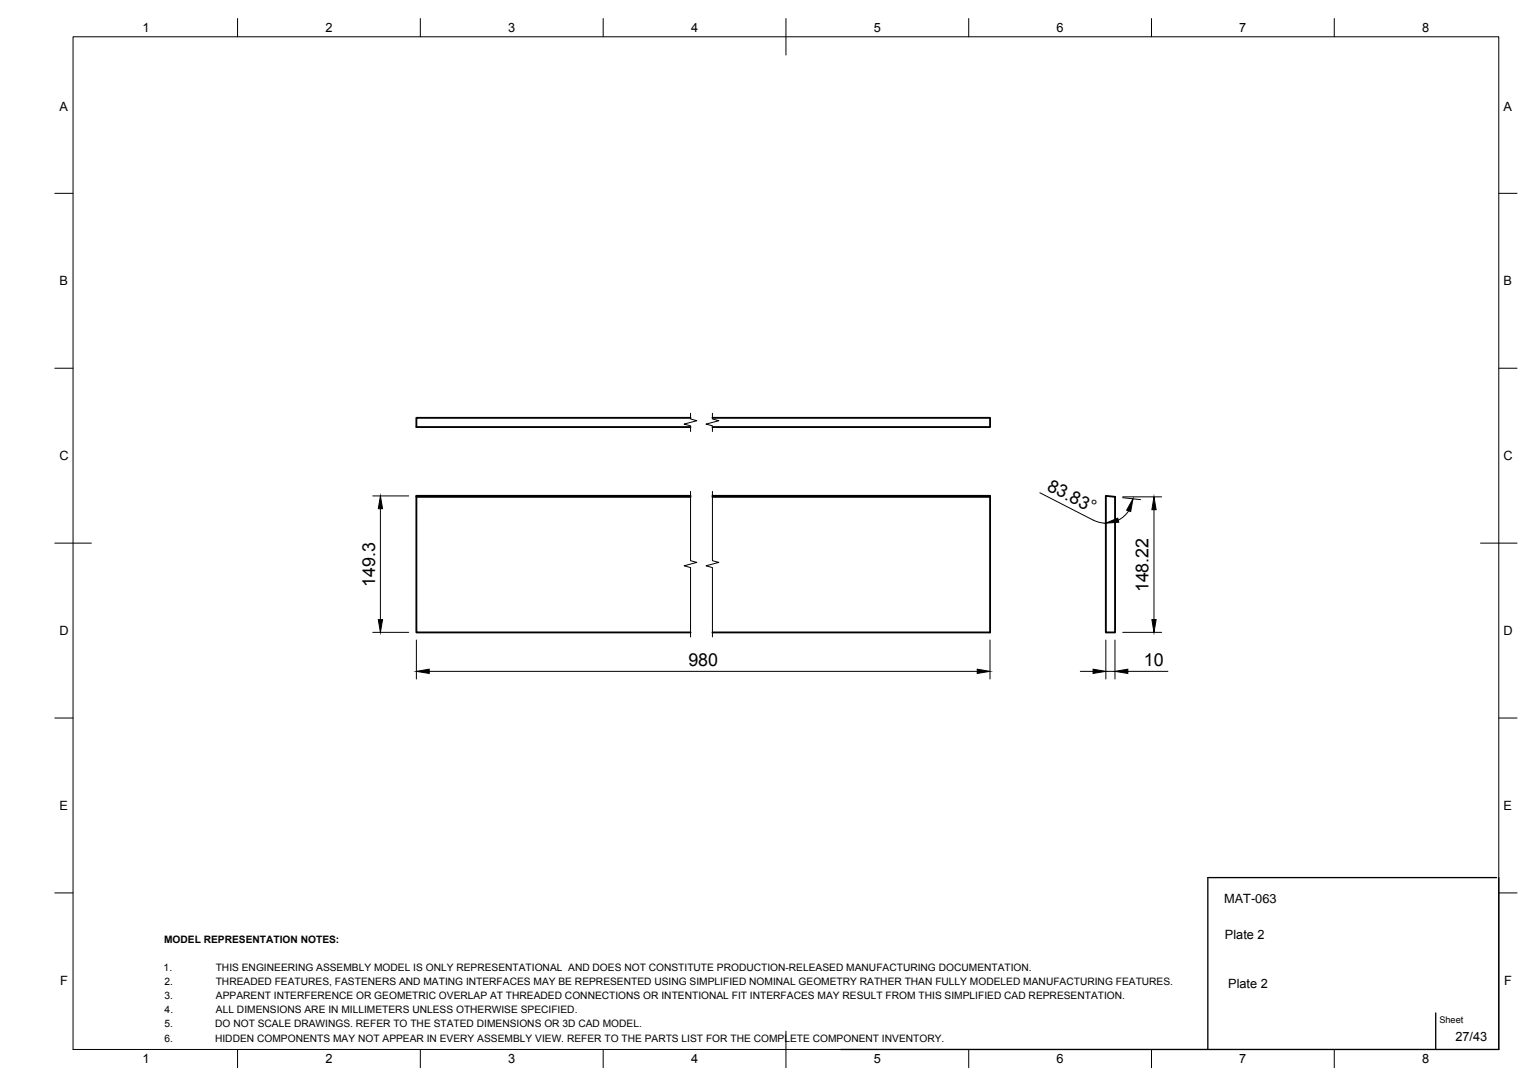
ISO-10303-21;
HEADER;
/* Generated by software containing ST-Developer
 * from STEP Tools, Inc. (www.steptools.com) 
 */

FILE_DESCRIPTION(
/* description */ (''),
/* implementation_level */ '2;1');

FILE_NAME(
/* name */ 'Plate 2.step',
/* time_stamp */ '2026-10-24T09:43:01-07:00',
/* author */ (''),
/* organization */ (''),
/* preprocessor_version */ 'ST-DEVELOPER v20.2',
/* originating_system */ 'Autodesk Translation Framework v15.15.0.0',
/* authorisation */ '');

FILE_SCHEMA (('AUTOMOTIVE_DESIGN { 1 0 10303 214 3 1 1 }'));
ENDSEC;

DATA;
#10=MECHANICAL_DESIGN_GEOMETRIC_PRESENTATION_REPRESENTATION('',(#292),#11112);
#226=SHAPE_REPRESENTATION_RELATIONSHIP('SRR','None',#11251,#259);
#259=ADVANCED_BREP_SHAPE_REPRESENTATION('',(#325),#11096);
#292=STYLED_ITEM('',(#11426),#325);
#325=MANIFOLD_SOLID_BREP('Plate 2',#6029);
#615=PLANE('',#7061);
#616=PLANE('',#7062);
#617=PLANE('',#7063);
#618=PLANE('',#7064);
#619=PLANE('',#7065);
#620=PLANE('',#7066);
#951=FACE_OUTER_BOUND('',#1435,.T.);
#952=FACE_OUTER_BOUND('',#1436,.T.);
#953=FACE_OUTER_BOUND('',#1437,.T.);
#954=FACE_OUTER_BOUND('',#1438,.T.);
#955=FACE_OUTER_BOUND('',#1439,.T.);
#956=FACE_OUTER_BOUND('',#1440,.T.);
#1435=EDGE_LOOP('',(#5149,#5150,#5151,#5152));
#1436=EDGE_LOOP('',(#5153,#5154,#5155,#5156));
#1437=EDGE_LOOP('',(#5157,#5158,#5159,#5160));
#1438=EDGE_LOOP('',(#5161,#5162,#5163,#5164));
#1439=EDGE_LOOP('',(#5165,#5166,#5167,#5168));
#1440=EDGE_LOOP('',(#5169,#5170,#5171,#5172));
#1810=LINE('',#10614,#2169);
#1811=LINE('',#10616,#2170);
#1812=LINE('',#10618,#2171);
#1813=LINE('',#10619,#2172);
#1814=LINE('',#10622,#2173);
#1815=LINE('',#10624,#2174);
#1816=LINE('',#10625,#2175);
#1817=LINE('',#10628,#2176);
#1818=LINE('',#10629,#2177);
#1819=LINE('',#10632,#2178);
#1820=LINE('',#10633,#2179);
#1821=LINE('',#10635,#2180);
#2169=VECTOR('',#8822,0.01);
#2170=VECTOR('',#8823,0.01);
#2171=VECTOR('',#8824,0.01);
#2172=VECTOR('',#8825,0.01);
#2173=VECTOR('',#8828,0.01);
#2174=VECTOR('',#8829,0.01);
#2175=VECTOR('',#8830,0.01);
#2176=VECTOR('',#8833,0.01);
#2177=VECTOR('',#8834,0.01);
#2178=VECTOR('',#8837,0.01);
#2179=VECTOR('',#8838,0.01);
#2180=VECTOR('',#8841,0.01);
#3062=VERTEX_POINT('',#10612);
#3063=VERTEX_POINT('',#10613);
#3064=VERTEX_POINT('',#10615);
#3065=VERTEX_POINT('',#10617);
#3066=VERTEX_POINT('',#10621);
#3067=VERTEX_POINT('',#10623);
#3068=VERTEX_POINT('',#10627);
#3069=VERTEX_POINT('',#10631);
#3778=EDGE_CURVE('',#3062,#3063,#1810,.T.);
#3779=EDGE_CURVE('',#3064,#3062,#1811,.T.);
#3780=EDGE_CURVE('',#3065,#3064,#1812,.T.);
#3781=EDGE_CURVE('',#3063,#3065,#1813,.T.);
#3782=EDGE_CURVE('',#3066,#3062,#1814,.T.);
#3783=EDGE_CURVE('',#3067,#3066,#1815,.T.);
#3784=EDGE_CURVE('',#3064,#3067,#1816,.T.);
#3785=EDGE_CURVE('',#3068,#3067,#1817,.T.);
#3786=EDGE_CURVE('',#3065,#3068,#1818,.T.);
#3787=EDGE_CURVE('',#3063,#3069,#1819,.T.);
#3788=EDGE_CURVE('',#3069,#3066,#1820,.T.);
#3789=EDGE_CURVE('',#3068,#3069,#1821,.T.);
#5149=ORIENTED_EDGE('',*,*,#3778,.F.);
#5150=ORIENTED_EDGE('',*,*,#3779,.F.);
#5151=ORIENTED_EDGE('',*,*,#3780,.F.);
#5152=ORIENTED_EDGE('',*,*,#3781,.F.);
#5153=ORIENTED_EDGE('',*,*,#3782,.F.);
#5154=ORIENTED_EDGE('',*,*,#3783,.F.);
#5155=ORIENTED_EDGE('',*,*,#3784,.F.);
#5156=ORIENTED_EDGE('',*,*,#3779,.T.);
#5157=ORIENTED_EDGE('',*,*,#3784,.T.);
#5158=ORIENTED_EDGE('',*,*,#3785,.F.);
#5159=ORIENTED_EDGE('',*,*,#3786,.F.);
#5160=ORIENTED_EDGE('',*,*,#3780,.T.);
#5161=ORIENTED_EDGE('',*,*,#3782,.T.);
#5162=ORIENTED_EDGE('',*,*,#3778,.T.);
#5163=ORIENTED_EDGE('',*,*,#3787,.T.);
#5164=ORIENTED_EDGE('',*,*,#3788,.T.);
#5165=ORIENTED_EDGE('',*,*,#3788,.F.);
#5166=ORIENTED_EDGE('',*,*,#3789,.F.);
#5167=ORIENTED_EDGE('',*,*,#3785,.T.);
#5168=ORIENTED_EDGE('',*,*,#3783,.T.);
#5169=ORIENTED_EDGE('',*,*,#3787,.F.);
#5170=ORIENTED_EDGE('',*,*,#3781,.T.);
#5171=ORIENTED_EDGE('',*,*,#3786,.T.);
#5172=ORIENTED_EDGE('',*,*,#3789,.T.);
#5924=ADVANCED_FACE('',(#951),#615,.F.);
#5925=ADVANCED_FACE('',(#952),#616,.F.);
#5926=ADVANCED_FACE('',(#953),#617,.F.);
#5927=ADVANCED_FACE('',(#954),#618,.T.);
#5928=ADVANCED_FACE('',(#955),#619,.F.);
#5929=ADVANCED_FACE('',(#956),#620,.F.);
#6029=CLOSED_SHELL('',(#5924,#5925,#5926,#5927,#5928,#5929));
#7060=AXIS2_PLACEMENT_3D('',#10610,#8818,#8819);
#7061=AXIS2_PLACEMENT_3D('',#10611,#8820,#8821);
#7062=AXIS2_PLACEMENT_3D('',#10620,#8826,#8827);
#7063=AXIS2_PLACEMENT_3D('',#10626,#8831,#8832);
#7064=AXIS2_PLACEMENT_3D('',#10630,#8835,#8836);
#7065=AXIS2_PLACEMENT_3D('',#10634,#8839,#8840);
#7066=AXIS2_PLACEMENT_3D('',#10636,#8842,#8843);
#8818=DIRECTION('axis',(0.,0.,1.));
#8819=DIRECTION('refdir',(1.,0.,0.));
#8820=DIRECTION('center_axis',(0.,0.,-1.));
#8821=DIRECTION('ref_axis',(-1.,0.,0.));
#8822=DIRECTION('',(0.,1.,0.));
#8823=DIRECTION('',(-1.,0.,0.));
#8824=DIRECTION('',(0.,-1.,0.));
#8825=DIRECTION('',(1.,0.,0.));
#8826=DIRECTION('center_axis',(-7.28280409740021E-18,1.,-6.81994143705154E-16));
#8827=DIRECTION('ref_axis',(-2.00053299278642E-49,6.81994143705154E-16,
1.));
#8828=DIRECTION('',(0.,0.,1.));
#8829=DIRECTION('',(-1.,0.,0.));
#8830=DIRECTION('',(0.,0.,-1.));
#8831=DIRECTION('center_axis',(-1.,-9.93231300437194E-17,-1.29261680723712E-15));
#8832=DIRECTION('ref_axis',(-1.29261680723712E-15,0.,1.));
#8833=DIRECTION('',(0.,-1.,0.));
#8834=DIRECTION('',(0.,-0.107473383594446,-0.994207962057618));
#8835=DIRECTION('center_axis',(-1.,9.93231300437194E-17,1.29261680723712E-15));
#8836=DIRECTION('ref_axis',(1.29261680723712E-15,0.,1.));
#8837=DIRECTION('',(0.,-0.107473383594446,-0.994207962057618));
#8838=DIRECTION('',(0.,-1.,0.));
#8839=DIRECTION('center_axis',(-2.10796718596837E-17,-1.82172040081484E-16,
1.));
#8840=DIRECTION('ref_axis',(0.,-1.,-1.82172040081484E-16));
#8841=DIRECTION('',(-1.,0.,0.));
#8842=DIRECTION('center_axis',(5.30402919874122E-18,-0.994207962057617,
0.107473383594448));
#8843=DIRECTION('ref_axis',(1.08940721566226E-34,-0.107473383594448,-0.994207962057617));
#10610=CARTESIAN_POINT('',(0.,0.,0.));
#10611=CARTESIAN_POINT('Origin',(-5.27355936696949E-17,-0.275347663,0.388147024999997));
#10612=CARTESIAN_POINT('',(-0.489999999999528,-0.349999999999892,0.38814702499999));
#10613=CARTESIAN_POINT('',(-0.489999999999528,-0.200695326000145,0.388147024999907));
#10614=CARTESIAN_POINT('',(-0.49,-0.349999999962674,0.388147024999997));
#10615=CARTESIAN_POINT('',(0.489999999999528,-0.349999999999892,0.38814702499999));
#10616=CARTESIAN_POINT('',(0.489999999755,-0.35,0.388147024999997));
#10617=CARTESIAN_POINT('',(0.489999999999528,-0.200695326000145,0.388147024999907));
#10618=CARTESIAN_POINT('',(0.49,-0.200695326040595,0.388147024999997));
#10619=CARTESIAN_POINT('',(-0.489999999755,-0.200695326,0.388147024999997));
#10620=CARTESIAN_POINT('Origin',(-5.27355936696949E-17,-0.35,0.383147025));
#10621=CARTESIAN_POINT('',(-0.489999999999528,-0.349999999999892,0.378147025000008));
#10622=CARTESIAN_POINT('',(-0.49,-0.35,0.3781470250025));
#10623=CARTESIAN_POINT('',(0.489999999999528,-0.349999999999892,0.378147025000008));
#10624=CARTESIAN_POINT('',(0.489999999755,-0.35,0.378147025));
#10625=CARTESIAN_POINT('',(0.49,-0.35,0.3881470249975));
#10626=CARTESIAN_POINT('Origin',(0.49,-0.275347663043444,0.383147025));
#10627=CARTESIAN_POINT('',(0.489999999999528,-0.201776321000629,0.378147024999632));
#10628=CARTESIAN_POINT('',(0.49,-0.201776321653339,0.378147025));
#10629=CARTESIAN_POINT('',(0.49,-0.200695326001004,0.388147024990716));
#10630=CARTESIAN_POINT('Origin',(-0.49,-0.275347663043444,0.383147025));
#10631=CARTESIAN_POINT('',(-0.489999999999528,-0.201776321000629,0.378147024999632));
#10632=CARTESIAN_POINT('',(-0.49,-0.200695326001004,0.388147024990716));
#10633=CARTESIAN_POINT('',(-0.49,-0.201776321653339,0.378147025));
#10634=CARTESIAN_POINT('Origin',(-6.68909372336657E-17,-0.2758881605,0.378147025000002));
#10635=CARTESIAN_POINT('',(0.489999999755,-0.201776321,0.378147025000002));
#10636=CARTESIAN_POINT('Origin',(-5.27355936696949E-17,-0.2012358235,0.383147025));
#11057=UNCERTAINTY_MEASURE_WITH_UNIT(LENGTH_MEASURE(1.E-5),#11113,
'DISTANCE_ACCURACY_VALUE',
'Maximum model space distance between geometric entities at asserted c
onnectivities');
#11073=UNCERTAINTY_MEASURE_WITH_UNIT(LENGTH_MEASURE(1.E-5),#11113,
'DISTANCE_ACCURACY_VALUE',
'Maximum model space distance between geometric entities at asserted c
onnectivities');
#11096=(
GEOMETRIC_REPRESENTATION_CONTEXT(3)
GLOBAL_UNCERTAINTY_ASSIGNED_CONTEXT((#11057))
GLOBAL_UNIT_ASSIGNED_CONTEXT((#11113,#11114,#11115))
REPRESENTATION_CONTEXT('','3D')
);
#11112=(
GEOMETRIC_REPRESENTATION_CONTEXT(3)
GLOBAL_UNCERTAINTY_ASSIGNED_CONTEXT((#11073))
GLOBAL_UNIT_ASSIGNED_CONTEXT((#11113,#11114,#11115))
REPRESENTATION_CONTEXT('','3D')
);
#11113=(
LENGTH_UNIT()
NAMED_UNIT(*)
SI_UNIT($,.METRE.)
);
#11114=(
NAMED_UNIT(*)
PLANE_ANGLE_UNIT()
SI_UNIT($,.RADIAN.)
);
#11115=(
NAMED_UNIT(*)
SI_UNIT($,.STERADIAN.)
SOLID_ANGLE_UNIT()
);
#11138=SHAPE_DEFINITION_REPRESENTATION(#11183,#11251);
#11183=PRODUCT_DEFINITION_SHAPE('',$,#11290);
#11251=SHAPE_REPRESENTATION('',(#7060),#11096);
#11267=PRODUCT_DEFINITION_CONTEXT('part definition',#11383,'design');
#11290=PRODUCT_DEFINITION('Plate 2','Plate 2',#11328,#11267);
#11328=PRODUCT_DEFINITION_FORMATION('',$,#11407);
#11383=APPLICATION_CONTEXT(
'Core Data for Automotive Mechanical Design Process');
#11384=PRODUCT_CONTEXT('part definition',#11383,'mechanical');
#11407=PRODUCT('Plate 2','Plate 2','all_plates__ DE     2307',(#11384));
#11426=PRESENTATION_STYLE_ASSIGNMENT((#11430));
#11430=SURFACE_STYLE_USAGE(.BOTH.,#11434);
#11434=SURFACE_SIDE_STYLE('',(#11438));
#11438=SURFACE_STYLE_FILL_AREA(#11442);
#11442=FILL_AREA_STYLE('Opaque(202,209,238)',(#11446));
#11446=FILL_AREA_STYLE_COLOUR('Opaque(202,209,238)',#11450);
#11450=COLOUR_RGB('Opaque(202,209,238)',0.792156862745098,0.819607843137255,
0.933333333333333);
ENDSEC;
END-ISO-10303-21;
